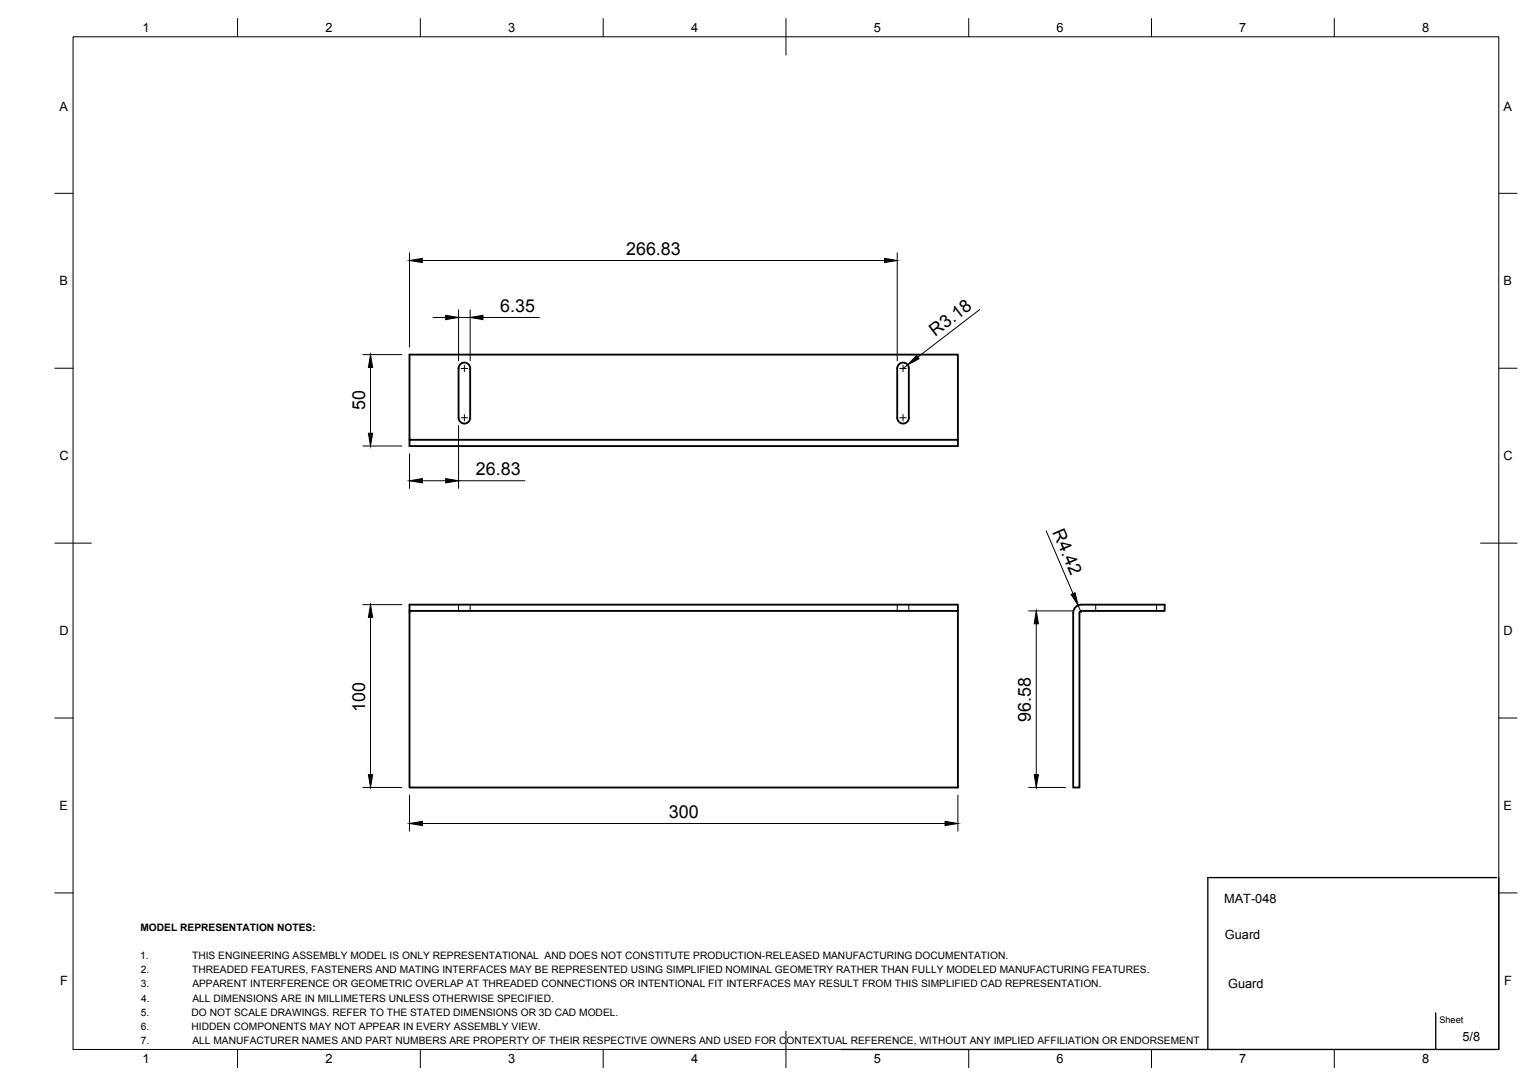
ISO-10303-21;
HEADER;
/* Generated by software containing ST-Developer
 * from STEP Tools, Inc. (www.steptools.com) 
 */

FILE_DESCRIPTION(
/* description */ ('STEP AP214'),
/* implementation_level */ '2;1');

FILE_NAME(
/* name */ 'Guard.step',
/* time_stamp */ '2026-11-14T22:24:45-08:00',
/* author */ (''),
/* organization */ (''),
/* preprocessor_version */ 'ST-DEVELOPER v20.2',
/* originating_system */ 'Autodesk Translation Framework v15.17.0.0',
/* authorisation */ '');

FILE_SCHEMA (('AUTOMOTIVE_DESIGN { 1 0 10303 214 3 1 1 }'));
ENDSEC;

DATA;
#10=MECHANICAL_DESIGN_GEOMETRIC_PRESENTATION_REPRESENTATION('',(#128),#5599);
#103=FACE_BOUND('',#588,.T.);
#104=FACE_BOUND('',#589,.T.);
#105=FACE_BOUND('',#592,.T.);
#106=FACE_BOUND('',#593,.T.);
#116=SHAPE_REPRESENTATION_RELATIONSHIP('SRR','None',#5644,#122);
#122=ADVANCED_BREP_SHAPE_REPRESENTATION('',(#134),#5596);
#128=STYLED_ITEM('',(#5680),#134);
#134=MANIFOLD_SOLID_BREP('Body1',#3310);
#171=CYLINDRICAL_SURFACE('',#3578,4.42);
#172=CYLINDRICAL_SURFACE('',#3582,1.);
#173=CYLINDRICAL_SURFACE('',#3585,3.17500000000003);
#174=CYLINDRICAL_SURFACE('',#3587,3.17500000000002);
#175=CYLINDRICAL_SURFACE('',#3589,3.17500000000004);
#176=CYLINDRICAL_SURFACE('',#3591,3.17500000000004);
#237=CIRCLE('',#3560,4.42);
#238=CIRCLE('',#3561,1.);
#239=CIRCLE('',#3564,4.42);
#240=CIRCLE('',#3565,1.);
#241=CIRCLE('',#3568,3.17500000000004);
#242=CIRCLE('',#3569,3.17500000000004);
#243=CIRCLE('',#3570,3.17500000000003);
#244=CIRCLE('',#3571,3.17500000000002);
#245=CIRCLE('',#3574,3.17500000000004);
#246=CIRCLE('',#3575,3.17500000000004);
#247=CIRCLE('',#3576,3.17500000000003);
#248=CIRCLE('',#3577,3.17500000000002);
#403=FACE_OUTER_BOUND('',#583,.T.);
#404=FACE_OUTER_BOUND('',#584,.T.);
#405=FACE_OUTER_BOUND('',#585,.T.);
#406=FACE_OUTER_BOUND('',#586,.T.);
#407=FACE_OUTER_BOUND('',#587,.T.);
#408=FACE_OUTER_BOUND('',#590,.T.);
#409=FACE_OUTER_BOUND('',#591,.T.);
#410=FACE_OUTER_BOUND('',#594,.T.);
#411=FACE_OUTER_BOUND('',#595,.T.);
#412=FACE_OUTER_BOUND('',#596,.T.);
#413=FACE_OUTER_BOUND('',#597,.T.);
#414=FACE_OUTER_BOUND('',#598,.T.);
#415=FACE_OUTER_BOUND('',#599,.T.);
#416=FACE_OUTER_BOUND('',#600,.T.);
#417=FACE_OUTER_BOUND('',#601,.T.);
#418=FACE_OUTER_BOUND('',#602,.T.);
#419=FACE_OUTER_BOUND('',#603,.T.);
#420=FACE_OUTER_BOUND('',#604,.T.);
#421=FACE_OUTER_BOUND('',#605,.T.);
#422=FACE_OUTER_BOUND('',#606,.T.);
#423=FACE_OUTER_BOUND('',#607,.T.);
#424=FACE_OUTER_BOUND('',#608,.T.);
#583=EDGE_LOOP('',(#2731,#2732,#2733,#2734));
#584=EDGE_LOOP('',(#2735,#2736,#2737,#2738));
#585=EDGE_LOOP('',(#2739,#2740,#2741,#2742));
#586=EDGE_LOOP('',(#2743,#2744,#2745,#2746));
#587=EDGE_LOOP('',(#2747,#2748,#2749,#2750));
#588=EDGE_LOOP('',(#2751,#2752,#2753,#2754));
#589=EDGE_LOOP('',(#2755,#2756,#2757,#2758));
#590=EDGE_LOOP('',(#2759,#2760,#2761,#2762));
#591=EDGE_LOOP('',(#2763,#2764,#2765,#2766));
#592=EDGE_LOOP('',(#2767,#2768,#2769,#2770));
#593=EDGE_LOOP('',(#2771,#2772,#2773,#2774));
#594=EDGE_LOOP('',(#2775,#2776,#2777,#2778));
#595=EDGE_LOOP('',(#2779,#2780,#2781,#2782));
#596=EDGE_LOOP('',(#2783,#2784,#2785,#2786));
#597=EDGE_LOOP('',(#2787,#2788,#2789,#2790));
#598=EDGE_LOOP('',(#2791,#2792,#2793,#2794));
#599=EDGE_LOOP('',(#2795,#2796,#2797,#2798));
#600=EDGE_LOOP('',(#2799,#2800,#2801,#2802));
#601=EDGE_LOOP('',(#2803,#2804,#2805,#2806));
#602=EDGE_LOOP('',(#2807,#2808,#2809,#2810));
#603=EDGE_LOOP('',(#2811,#2812,#2813,#2814));
#604=EDGE_LOOP('',(#2815,#2816,#2817,#2818));
#605=EDGE_LOOP('',(#2819,#2820,#2821,#2822));
#606=EDGE_LOOP('',(#2823,#2824,#2825,#2826));
#607=EDGE_LOOP('',(#2827,#2828,#2829,#2830));
#608=EDGE_LOOP('',(#2831,#2832,#2833,#2834));
#911=LINE('',#5285,#1267);
#912=LINE('',#5289,#1268);
#913=LINE('',#5293,#1269);
#914=LINE('',#5295,#1270);
#915=LINE('',#5296,#1271);
#916=LINE('',#5300,#1272);
#917=LINE('',#5304,#1273);
#918=LINE('',#5308,#1274);
#919=LINE('',#5310,#1275);
#920=LINE('',#5311,#1276);
#921=LINE('',#5314,#1277);
#922=LINE('',#5315,#1278);
#923=LINE('',#5316,#1279);
#924=LINE('',#5319,#1280);
#925=LINE('',#5323,#1281);
#926=LINE('',#5327,#1282);
#927=LINE('',#5331,#1283);
#928=LINE('',#5335,#1284);
#929=LINE('',#5336,#1285);
#930=LINE('',#5338,#1286);
#931=LINE('',#5339,#1287);
#932=LINE('',#5344,#1288);
#933=LINE('',#5347,#1289);
#934=LINE('',#5352,#1290);
#935=LINE('',#5355,#1291);
#936=LINE('',#5357,#1292);
#937=LINE('',#5360,#1293);
#938=LINE('',#5361,#1294);
#939=LINE('',#5364,#1295);
#940=LINE('',#5365,#1296);
#941=LINE('',#5367,#1297);
#942=LINE('',#5368,#1298);
#943=LINE('',#5373,#1299);
#944=LINE('',#5374,#1300);
#945=LINE('',#5376,#1301);
#946=LINE('',#5378,#1302);
#947=LINE('',#5381,#1303);
#948=LINE('',#5382,#1304);
#949=LINE('',#5384,#1305);
#950=LINE('',#5386,#1306);
#1267=VECTOR('',#4305,1000.);
#1268=VECTOR('',#4308,1000.);
#1269=VECTOR('',#4313,1000.);
#1270=VECTOR('',#4314,1000.);
#1271=VECTOR('',#4315,1000.);
#1272=VECTOR('',#4318,1000.);
#1273=VECTOR('',#4321,1000.);
#1274=VECTOR('',#4326,1000.);
#1275=VECTOR('',#4327,1000.);
#1276=VECTOR('',#4328,1000.);
#1277=VECTOR('',#4331,1000.);
#1278=VECTOR('',#4332,1000.);
#1279=VECTOR('',#4333,1000.);
#1280=VECTOR('',#4334,1000.);
#1281=VECTOR('',#4337,1000.);
#1282=VECTOR('',#4340,1000.);
#1283=VECTOR('',#4343,1000.);
#1284=VECTOR('',#4348,1000.);
#1285=VECTOR('',#4349,1000.);
#1286=VECTOR('',#4352,1000.);
#1287=VECTOR('',#4353,1000.);
#1288=VECTOR('',#4356,1000.);
#1289=VECTOR('',#4359,1000.);
#1290=VECTOR('',#4362,1000.);
#1291=VECTOR('',#4365,1000.);
#1292=VECTOR('',#4368,1000.);
#1293=VECTOR('',#4371,1000.);
#1294=VECTOR('',#4372,1000.);
#1295=VECTOR('',#4375,1000.);
#1296=VECTOR('',#4376,1000.);
#1297=VECTOR('',#4379,1000.);
#1298=VECTOR('',#4380,1000.);
#1299=VECTOR('',#4389,1000.);
#1300=VECTOR('',#4390,1000.);
#1301=VECTOR('',#4393,1000.);
#1302=VECTOR('',#4396,1000.);
#1303=VECTOR('',#4401,1000.);
#1304=VECTOR('',#4402,1000.);
#1305=VECTOR('',#4405,1000.);
#1306=VECTOR('',#4408,1000.);
#1559=VERTEX_POINT('',#5283);
#1560=VERTEX_POINT('',#5284);
#1561=VERTEX_POINT('',#5286);
#1562=VERTEX_POINT('',#5288);
#1563=VERTEX_POINT('',#5292);
#1564=VERTEX_POINT('',#5294);
#1565=VERTEX_POINT('',#5298);
#1566=VERTEX_POINT('',#5299);
#1567=VERTEX_POINT('',#5301);
#1568=VERTEX_POINT('',#5303);
#1569=VERTEX_POINT('',#5307);
#1570=VERTEX_POINT('',#5309);
#1571=VERTEX_POINT('',#5313);
#1572=VERTEX_POINT('',#5317);
#1573=VERTEX_POINT('',#5318);
#1574=VERTEX_POINT('',#5320);
#1575=VERTEX_POINT('',#5322);
#1576=VERTEX_POINT('',#5325);
#1577=VERTEX_POINT('',#5326);
#1578=VERTEX_POINT('',#5328);
#1579=VERTEX_POINT('',#5330);
#1580=VERTEX_POINT('',#5334);
#1581=VERTEX_POINT('',#5340);
#1582=VERTEX_POINT('',#5341);
#1583=VERTEX_POINT('',#5343);
#1584=VERTEX_POINT('',#5345);
#1585=VERTEX_POINT('',#5348);
#1586=VERTEX_POINT('',#5349);
#1587=VERTEX_POINT('',#5351);
#1588=VERTEX_POINT('',#5353);
#1589=VERTEX_POINT('',#5359);
#1590=VERTEX_POINT('',#5363);
#1963=EDGE_CURVE('',#1559,#1560,#911,.T.);
#1964=EDGE_CURVE('',#1561,#1559,#237,.T.);
#1965=EDGE_CURVE('',#1562,#1561,#912,.T.);
#1966=EDGE_CURVE('',#1562,#1560,#238,.T.);
#1967=EDGE_CURVE('',#1559,#1563,#913,.T.);
#1968=EDGE_CURVE('',#1560,#1564,#914,.T.);
#1969=EDGE_CURVE('',#1563,#1564,#915,.T.);
#1970=EDGE_CURVE('',#1565,#1566,#916,.T.);
#1971=EDGE_CURVE('',#1565,#1567,#239,.T.);
#1972=EDGE_CURVE('',#1568,#1567,#917,.T.);
#1973=EDGE_CURVE('',#1566,#1568,#240,.T.);
#1974=EDGE_CURVE('',#1569,#1565,#918,.T.);
#1975=EDGE_CURVE('',#1570,#1566,#919,.T.);
#1976=EDGE_CURVE('',#1570,#1569,#920,.T.);
#1977=EDGE_CURVE('',#1568,#1571,#921,.T.);
#1978=EDGE_CURVE('',#1564,#1571,#922,.T.);
#1979=EDGE_CURVE('',#1560,#1568,#923,.T.);
#1980=EDGE_CURVE('',#1572,#1573,#924,.T.);
#1981=EDGE_CURVE('',#1573,#1574,#241,.T.);
#1982=EDGE_CURVE('',#1574,#1575,#925,.T.);
#1983=EDGE_CURVE('',#1575,#1572,#242,.T.);
#1984=EDGE_CURVE('',#1576,#1577,#926,.T.);
#1985=EDGE_CURVE('',#1577,#1578,#243,.T.);
#1986=EDGE_CURVE('',#1578,#1579,#927,.T.);
#1987=EDGE_CURVE('',#1579,#1576,#244,.T.);
#1988=EDGE_CURVE('',#1580,#1571,#928,.T.);
#1989=EDGE_CURVE('',#1563,#1580,#929,.T.);
#1990=EDGE_CURVE('',#1567,#1580,#930,.T.);
#1991=EDGE_CURVE('',#1559,#1567,#931,.T.);
#1992=EDGE_CURVE('',#1581,#1582,#245,.T.);
#1993=EDGE_CURVE('',#1583,#1581,#932,.T.);
#1994=EDGE_CURVE('',#1584,#1583,#246,.T.);
#1995=EDGE_CURVE('',#1582,#1584,#933,.T.);
#1996=EDGE_CURVE('',#1585,#1586,#247,.T.);
#1997=EDGE_CURVE('',#1587,#1585,#934,.T.);
#1998=EDGE_CURVE('',#1588,#1587,#248,.T.);
#1999=EDGE_CURVE('',#1586,#1588,#935,.T.);
#2000=EDGE_CURVE('',#1561,#1565,#936,.T.);
#2001=EDGE_CURVE('',#1589,#1569,#937,.T.);
#2002=EDGE_CURVE('',#1589,#1561,#938,.T.);
#2003=EDGE_CURVE('',#1590,#1570,#939,.T.);
#2004=EDGE_CURVE('',#1590,#1589,#940,.T.);
#2005=EDGE_CURVE('',#1562,#1566,#941,.T.);
#2006=EDGE_CURVE('',#1590,#1562,#942,.T.);
#2007=EDGE_CURVE('',#1577,#1585,#943,.T.);
#2008=EDGE_CURVE('',#1578,#1586,#944,.T.);
#2009=EDGE_CURVE('',#1576,#1587,#945,.T.);
#2010=EDGE_CURVE('',#1579,#1588,#946,.T.);
#2011=EDGE_CURVE('',#1573,#1581,#947,.T.);
#2012=EDGE_CURVE('',#1574,#1582,#948,.T.);
#2013=EDGE_CURVE('',#1572,#1583,#949,.T.);
#2014=EDGE_CURVE('',#1575,#1584,#950,.T.);
#2731=ORIENTED_EDGE('',*,*,#1963,.F.);
#2732=ORIENTED_EDGE('',*,*,#1964,.F.);
#2733=ORIENTED_EDGE('',*,*,#1965,.F.);
#2734=ORIENTED_EDGE('',*,*,#1966,.T.);
#2735=ORIENTED_EDGE('',*,*,#1967,.F.);
#2736=ORIENTED_EDGE('',*,*,#1963,.T.);
#2737=ORIENTED_EDGE('',*,*,#1968,.T.);
#2738=ORIENTED_EDGE('',*,*,#1969,.F.);
#2739=ORIENTED_EDGE('',*,*,#1970,.F.);
#2740=ORIENTED_EDGE('',*,*,#1971,.T.);
#2741=ORIENTED_EDGE('',*,*,#1972,.F.);
#2742=ORIENTED_EDGE('',*,*,#1973,.F.);
#2743=ORIENTED_EDGE('',*,*,#1974,.T.);
#2744=ORIENTED_EDGE('',*,*,#1970,.T.);
#2745=ORIENTED_EDGE('',*,*,#1975,.F.);
#2746=ORIENTED_EDGE('',*,*,#1976,.T.);
#2747=ORIENTED_EDGE('',*,*,#1977,.T.);
#2748=ORIENTED_EDGE('',*,*,#1978,.F.);
#2749=ORIENTED_EDGE('',*,*,#1968,.F.);
#2750=ORIENTED_EDGE('',*,*,#1979,.T.);
#2751=ORIENTED_EDGE('',*,*,#1980,.T.);
#2752=ORIENTED_EDGE('',*,*,#1981,.T.);
#2753=ORIENTED_EDGE('',*,*,#1982,.T.);
#2754=ORIENTED_EDGE('',*,*,#1983,.T.);
#2755=ORIENTED_EDGE('',*,*,#1984,.T.);
#2756=ORIENTED_EDGE('',*,*,#1985,.T.);
#2757=ORIENTED_EDGE('',*,*,#1986,.T.);
#2758=ORIENTED_EDGE('',*,*,#1987,.T.);
#2759=ORIENTED_EDGE('',*,*,#1988,.F.);
#2760=ORIENTED_EDGE('',*,*,#1989,.F.);
#2761=ORIENTED_EDGE('',*,*,#1969,.T.);
#2762=ORIENTED_EDGE('',*,*,#1978,.T.);
#2763=ORIENTED_EDGE('',*,*,#1990,.F.);
#2764=ORIENTED_EDGE('',*,*,#1991,.F.);
#2765=ORIENTED_EDGE('',*,*,#1967,.T.);
#2766=ORIENTED_EDGE('',*,*,#1989,.T.);
#2767=ORIENTED_EDGE('',*,*,#1992,.F.);
#2768=ORIENTED_EDGE('',*,*,#1993,.F.);
#2769=ORIENTED_EDGE('',*,*,#1994,.F.);
#2770=ORIENTED_EDGE('',*,*,#1995,.F.);
#2771=ORIENTED_EDGE('',*,*,#1996,.F.);
#2772=ORIENTED_EDGE('',*,*,#1997,.F.);
#2773=ORIENTED_EDGE('',*,*,#1998,.F.);
#2774=ORIENTED_EDGE('',*,*,#1999,.F.);
#2775=ORIENTED_EDGE('',*,*,#1971,.F.);
#2776=ORIENTED_EDGE('',*,*,#2000,.F.);
#2777=ORIENTED_EDGE('',*,*,#1964,.T.);
#2778=ORIENTED_EDGE('',*,*,#1991,.T.);
#2779=ORIENTED_EDGE('',*,*,#1974,.F.);
#2780=ORIENTED_EDGE('',*,*,#2001,.F.);
#2781=ORIENTED_EDGE('',*,*,#2002,.T.);
#2782=ORIENTED_EDGE('',*,*,#2000,.T.);
#2783=ORIENTED_EDGE('',*,*,#1976,.F.);
#2784=ORIENTED_EDGE('',*,*,#2003,.F.);
#2785=ORIENTED_EDGE('',*,*,#2004,.T.);
#2786=ORIENTED_EDGE('',*,*,#2001,.T.);
#2787=ORIENTED_EDGE('',*,*,#1975,.T.);
#2788=ORIENTED_EDGE('',*,*,#2005,.F.);
#2789=ORIENTED_EDGE('',*,*,#2006,.F.);
#2790=ORIENTED_EDGE('',*,*,#2003,.T.);
#2791=ORIENTED_EDGE('',*,*,#1973,.T.);
#2792=ORIENTED_EDGE('',*,*,#1979,.F.);
#2793=ORIENTED_EDGE('',*,*,#1966,.F.);
#2794=ORIENTED_EDGE('',*,*,#2005,.T.);
#2795=ORIENTED_EDGE('',*,*,#2006,.T.);
#2796=ORIENTED_EDGE('',*,*,#1965,.T.);
#2797=ORIENTED_EDGE('',*,*,#2002,.F.);
#2798=ORIENTED_EDGE('',*,*,#2004,.F.);
#2799=ORIENTED_EDGE('',*,*,#1977,.F.);
#2800=ORIENTED_EDGE('',*,*,#1972,.T.);
#2801=ORIENTED_EDGE('',*,*,#1990,.T.);
#2802=ORIENTED_EDGE('',*,*,#1988,.T.);
#2803=ORIENTED_EDGE('',*,*,#2007,.T.);
#2804=ORIENTED_EDGE('',*,*,#1996,.T.);
#2805=ORIENTED_EDGE('',*,*,#2008,.F.);
#2806=ORIENTED_EDGE('',*,*,#1985,.F.);
#2807=ORIENTED_EDGE('',*,*,#2009,.T.);
#2808=ORIENTED_EDGE('',*,*,#1997,.T.);
#2809=ORIENTED_EDGE('',*,*,#2007,.F.);
#2810=ORIENTED_EDGE('',*,*,#1984,.F.);
#2811=ORIENTED_EDGE('',*,*,#2010,.T.);
#2812=ORIENTED_EDGE('',*,*,#1998,.T.);
#2813=ORIENTED_EDGE('',*,*,#2009,.F.);
#2814=ORIENTED_EDGE('',*,*,#1987,.F.);
#2815=ORIENTED_EDGE('',*,*,#2008,.T.);
#2816=ORIENTED_EDGE('',*,*,#1999,.T.);
#2817=ORIENTED_EDGE('',*,*,#2010,.F.);
#2818=ORIENTED_EDGE('',*,*,#1986,.F.);
#2819=ORIENTED_EDGE('',*,*,#2011,.T.);
#2820=ORIENTED_EDGE('',*,*,#1992,.T.);
#2821=ORIENTED_EDGE('',*,*,#2012,.F.);
#2822=ORIENTED_EDGE('',*,*,#1981,.F.);
#2823=ORIENTED_EDGE('',*,*,#2013,.T.);
#2824=ORIENTED_EDGE('',*,*,#1993,.T.);
#2825=ORIENTED_EDGE('',*,*,#2011,.F.);
#2826=ORIENTED_EDGE('',*,*,#1980,.F.);
#2827=ORIENTED_EDGE('',*,*,#2014,.T.);
#2828=ORIENTED_EDGE('',*,*,#1994,.T.);
#2829=ORIENTED_EDGE('',*,*,#2013,.F.);
#2830=ORIENTED_EDGE('',*,*,#1983,.F.);
#2831=ORIENTED_EDGE('',*,*,#2012,.T.);
#2832=ORIENTED_EDGE('',*,*,#1995,.T.);
#2833=ORIENTED_EDGE('',*,*,#2014,.F.);
#2834=ORIENTED_EDGE('',*,*,#1982,.F.);
#3099=PLANE('',#3559);
#3100=PLANE('',#3562);
#3101=PLANE('',#3563);
#3102=PLANE('',#3566);
#3103=PLANE('',#3567);
#3104=PLANE('',#3572);
#3105=PLANE('',#3573);
#3106=PLANE('',#3579);
#3107=PLANE('',#3580);
#3108=PLANE('',#3581);
#3109=PLANE('',#3583);
#3110=PLANE('',#3584);
#3111=PLANE('',#3586);
#3112=PLANE('',#3588);
#3113=PLANE('',#3590);
#3114=PLANE('',#3592);
#3253=ADVANCED_FACE('',(#403),#3099,.T.);
#3254=ADVANCED_FACE('',(#404),#3100,.T.);
#3255=ADVANCED_FACE('',(#405),#3101,.T.);
#3256=ADVANCED_FACE('',(#406),#3102,.T.);
#3257=ADVANCED_FACE('',(#407,#103,#104),#3103,.F.);
#3258=ADVANCED_FACE('',(#408),#3104,.T.);
#3259=ADVANCED_FACE('',(#409,#105,#106),#3105,.T.);
#3260=ADVANCED_FACE('',(#410),#171,.T.);
#3261=ADVANCED_FACE('',(#411),#3106,.T.);
#3262=ADVANCED_FACE('',(#412),#3107,.T.);
#3263=ADVANCED_FACE('',(#413),#3108,.F.);
#3264=ADVANCED_FACE('',(#414),#172,.F.);
#3265=ADVANCED_FACE('',(#415),#3109,.T.);
#3266=ADVANCED_FACE('',(#416),#3110,.F.);
#3267=ADVANCED_FACE('',(#417),#173,.F.);
#3268=ADVANCED_FACE('',(#418),#3111,.F.);
#3269=ADVANCED_FACE('',(#419),#174,.F.);
#3270=ADVANCED_FACE('',(#420),#3112,.F.);
#3271=ADVANCED_FACE('',(#421),#175,.F.);
#3272=ADVANCED_FACE('',(#422),#3113,.F.);
#3273=ADVANCED_FACE('',(#423),#176,.F.);
#3274=ADVANCED_FACE('',(#424),#3114,.F.);
#3310=CLOSED_SHELL('',(#3253,#3254,#3255,#3256,#3257,#3258,#3259,#3260,
#3261,#3262,#3263,#3264,#3265,#3266,#3267,#3268,#3269,#3270,#3271,#3272,
#3273,#3274));
#3558=AXIS2_PLACEMENT_3D('',#5281,#4301,#4302);
#3559=AXIS2_PLACEMENT_3D('',#5282,#4303,#4304);
#3560=AXIS2_PLACEMENT_3D('',#5287,#4306,#4307);
#3561=AXIS2_PLACEMENT_3D('',#5290,#4309,#4310);
#3562=AXIS2_PLACEMENT_3D('',#5291,#4311,#4312);
#3563=AXIS2_PLACEMENT_3D('',#5297,#4316,#4317);
#3564=AXIS2_PLACEMENT_3D('',#5302,#4319,#4320);
#3565=AXIS2_PLACEMENT_3D('',#5305,#4322,#4323);
#3566=AXIS2_PLACEMENT_3D('',#5306,#4324,#4325);
#3567=AXIS2_PLACEMENT_3D('',#5312,#4329,#4330);
#3568=AXIS2_PLACEMENT_3D('',#5321,#4335,#4336);
#3569=AXIS2_PLACEMENT_3D('',#5324,#4338,#4339);
#3570=AXIS2_PLACEMENT_3D('',#5329,#4341,#4342);
#3571=AXIS2_PLACEMENT_3D('',#5332,#4344,#4345);
#3572=AXIS2_PLACEMENT_3D('',#5333,#4346,#4347);
#3573=AXIS2_PLACEMENT_3D('',#5337,#4350,#4351);
#3574=AXIS2_PLACEMENT_3D('',#5342,#4354,#4355);
#3575=AXIS2_PLACEMENT_3D('',#5346,#4357,#4358);
#3576=AXIS2_PLACEMENT_3D('',#5350,#4360,#4361);
#3577=AXIS2_PLACEMENT_3D('',#5354,#4363,#4364);
#3578=AXIS2_PLACEMENT_3D('',#5356,#4366,#4367);
#3579=AXIS2_PLACEMENT_3D('',#5358,#4369,#4370);
#3580=AXIS2_PLACEMENT_3D('',#5362,#4373,#4374);
#3581=AXIS2_PLACEMENT_3D('',#5366,#4377,#4378);
#3582=AXIS2_PLACEMENT_3D('',#5369,#4381,#4382);
#3583=AXIS2_PLACEMENT_3D('',#5370,#4383,#4384);
#3584=AXIS2_PLACEMENT_3D('',#5371,#4385,#4386);
#3585=AXIS2_PLACEMENT_3D('',#5372,#4387,#4388);
#3586=AXIS2_PLACEMENT_3D('',#5375,#4391,#4392);
#3587=AXIS2_PLACEMENT_3D('',#5377,#4394,#4395);
#3588=AXIS2_PLACEMENT_3D('',#5379,#4397,#4398);
#3589=AXIS2_PLACEMENT_3D('',#5380,#4399,#4400);
#3590=AXIS2_PLACEMENT_3D('',#5383,#4403,#4404);
#3591=AXIS2_PLACEMENT_3D('',#5385,#4406,#4407);
#3592=AXIS2_PLACEMENT_3D('',#5387,#4409,#4410);
#4301=DIRECTION('axis',(0.,0.,1.));
#4302=DIRECTION('refdir',(1.,0.,0.));
#4303=DIRECTION('center_axis',(0.,0.,1.));
#4304=DIRECTION('ref_axis',(1.,0.,0.));
#4305=DIRECTION('',(0.,-1.,0.));
#4306=DIRECTION('center_axis',(0.,0.,-1.));
#4307=DIRECTION('ref_axis',(1.,0.,0.));
#4308=DIRECTION('',(-1.,-1.21734980770302E-14,0.));
#4309=DIRECTION('center_axis',(0.,0.,-1.));
#4310=DIRECTION('ref_axis',(1.,0.,0.));
#4311=DIRECTION('center_axis',(0.,0.,1.));
#4312=DIRECTION('ref_axis',(1.,0.,0.));
#4313=DIRECTION('',(1.,0.,0.));
#4314=DIRECTION('',(1.,0.,0.));
#4315=DIRECTION('',(0.,-1.,0.));
#4316=DIRECTION('center_axis',(0.,0.,-1.));
#4317=DIRECTION('ref_axis',(-1.,0.,0.));
#4318=DIRECTION('',(1.,1.21734980770302E-14,0.));
#4319=DIRECTION('center_axis',(0.,0.,-1.));
#4320=DIRECTION('ref_axis',(1.,0.,0.));
#4321=DIRECTION('',(0.,1.,0.));
#4322=DIRECTION('center_axis',(0.,0.,-1.));
#4323=DIRECTION('ref_axis',(1.,0.,0.));
#4324=DIRECTION('center_axis',(0.,0.,-1.));
#4325=DIRECTION('ref_axis',(-1.,0.,0.));
#4326=DIRECTION('',(0.,1.,0.));
#4327=DIRECTION('',(0.,1.,0.));
#4328=DIRECTION('',(-1.,0.,0.));
#4329=DIRECTION('center_axis',(0.,1.,0.));
#4330=DIRECTION('ref_axis',(0.,0.,1.));
#4331=DIRECTION('',(1.,0.,0.));
#4332=DIRECTION('',(0.,0.,-1.));
#4333=DIRECTION('',(0.,0.,-1.));
#4334=DIRECTION('',(1.,0.,0.));
#4335=DIRECTION('center_axis',(0.,1.,0.));
#4336=DIRECTION('ref_axis',(0.,0.,1.));
#4337=DIRECTION('',(-1.,0.,0.));
#4338=DIRECTION('center_axis',(0.,1.,0.));
#4339=DIRECTION('ref_axis',(0.,0.,1.));
#4340=DIRECTION('',(1.,0.,0.));
#4341=DIRECTION('center_axis',(0.,1.,0.));
#4342=DIRECTION('ref_axis',(0.,0.,1.));
#4343=DIRECTION('',(-1.,0.,5.14311353474695E-16));
#4344=DIRECTION('center_axis',(0.,1.,0.));
#4345=DIRECTION('ref_axis',(0.,0.,1.));
#4346=DIRECTION('center_axis',(1.,0.,0.));
#4347=DIRECTION('ref_axis',(0.,0.,-1.));
#4348=DIRECTION('',(0.,-1.,0.));
#4349=DIRECTION('',(0.,0.,-1.));
#4350=DIRECTION('center_axis',(0.,1.,0.));
#4351=DIRECTION('ref_axis',(0.,0.,1.));
#4352=DIRECTION('',(1.,0.,0.));
#4353=DIRECTION('',(0.,0.,-1.));
#4354=DIRECTION('center_axis',(0.,1.,0.));
#4355=DIRECTION('ref_axis',(0.,0.,1.));
#4356=DIRECTION('',(1.,0.,0.));
#4357=DIRECTION('center_axis',(0.,1.,0.));
#4358=DIRECTION('ref_axis',(0.,0.,1.));
#4359=DIRECTION('',(-1.,0.,0.));
#4360=DIRECTION('center_axis',(0.,1.,0.));
#4361=DIRECTION('ref_axis',(0.,0.,-1.));
#4362=DIRECTION('',(1.,0.,0.));
#4363=DIRECTION('center_axis',(0.,1.,0.));
#4364=DIRECTION('ref_axis',(0.,0.,-1.));
#4365=DIRECTION('',(-1.,0.,5.14311353474694E-16));
#4366=DIRECTION('center_axis',(0.,0.,-1.));
#4367=DIRECTION('ref_axis',(-1.,0.,0.));
#4368=DIRECTION('',(0.,0.,-1.));
#4369=DIRECTION('center_axis',(-1.,0.,0.));
#4370=DIRECTION('ref_axis',(0.,0.,1.));
#4371=DIRECTION('',(0.,0.,-1.));
#4372=DIRECTION('',(0.,1.,0.));
#4373=DIRECTION('center_axis',(0.,-1.,0.));
#4374=DIRECTION('ref_axis',(0.,0.,-1.));
#4375=DIRECTION('',(0.,0.,-1.));
#4376=DIRECTION('',(-1.,0.,0.));
#4377=DIRECTION('center_axis',(-1.,0.,0.));
#4378=DIRECTION('ref_axis',(0.,0.,1.));
#4379=DIRECTION('',(0.,0.,-1.));
#4380=DIRECTION('',(0.,1.,0.));
#4381=DIRECTION('center_axis',(0.,0.,-1.));
#4382=DIRECTION('ref_axis',(-1.,0.,0.));
#4383=DIRECTION('center_axis',(0.,0.,1.));
#4384=DIRECTION('ref_axis',(1.,0.,0.));
#4385=DIRECTION('center_axis',(0.,0.,1.));
#4386=DIRECTION('ref_axis',(1.,0.,0.));
#4387=DIRECTION('center_axis',(0.,1.,0.));
#4388=DIRECTION('ref_axis',(0.,0.,1.));
#4389=DIRECTION('',(0.,1.,0.));
#4390=DIRECTION('',(0.,1.,0.));
#4391=DIRECTION('center_axis',(0.,0.,1.));
#4392=DIRECTION('ref_axis',(1.,0.,0.));
#4393=DIRECTION('',(0.,1.,0.));
#4394=DIRECTION('center_axis',(0.,1.,0.));
#4395=DIRECTION('ref_axis',(0.,0.,1.));
#4396=DIRECTION('',(0.,1.,0.));
#4397=DIRECTION('center_axis',(-5.14311353474695E-16,0.,-1.));
#4398=DIRECTION('ref_axis',(-1.,0.,5.14311353474695E-16));
#4399=DIRECTION('center_axis',(0.,1.,0.));
#4400=DIRECTION('ref_axis',(0.,0.,1.));
#4401=DIRECTION('',(0.,1.,0.));
#4402=DIRECTION('',(0.,1.,0.));
#4403=DIRECTION('center_axis',(0.,0.,1.));
#4404=DIRECTION('ref_axis',(1.,0.,0.));
#4405=DIRECTION('',(0.,1.,0.));
#4406=DIRECTION('center_axis',(0.,1.,0.));
#4407=DIRECTION('ref_axis',(0.,0.,1.));
#4408=DIRECTION('',(0.,1.,0.));
#4409=DIRECTION('center_axis',(0.,0.,-1.));
#4410=DIRECTION('ref_axis',(-1.,0.,0.));
#5281=CARTESIAN_POINT('',(0.,0.,0.));
#5282=CARTESIAN_POINT('Origin',(4.42,100.,300.));
#5283=CARTESIAN_POINT('',(4.42,100.,300.));
#5284=CARTESIAN_POINT('',(4.42,96.58,300.));
#5285=CARTESIAN_POINT('',(4.42,100.,300.));
#5286=CARTESIAN_POINT('',(0.,95.5799999999999,300.));
#5287=CARTESIAN_POINT('Origin',(4.42,95.58,300.));
#5288=CARTESIAN_POINT('',(3.42,95.58,300.));
#5289=CARTESIAN_POINT('',(3.42,95.58,300.));
#5290=CARTESIAN_POINT('Origin',(4.42,95.58,300.));
#5291=CARTESIAN_POINT('Origin',(3.42,95.58,300.));
#5292=CARTESIAN_POINT('',(50.,100.,300.));
#5293=CARTESIAN_POINT('',(0.,100.,300.));
#5294=CARTESIAN_POINT('',(50.,96.58,300.));
#5295=CARTESIAN_POINT('',(0.,96.58,300.));
#5296=CARTESIAN_POINT('',(50.,100.,300.));
#5297=CARTESIAN_POINT('Origin',(0.,95.5799999999999,0.));
#5298=CARTESIAN_POINT('',(0.,95.5799999999999,0.));
#5299=CARTESIAN_POINT('',(3.42,95.58,-5.55111512312578E-14));
#5300=CARTESIAN_POINT('',(0.,95.5799999999999,0.));
#5301=CARTESIAN_POINT('',(4.42,100.,0.));
#5302=CARTESIAN_POINT('Origin',(4.42,95.58,0.));
#5303=CARTESIAN_POINT('',(4.42,96.58,0.));
#5304=CARTESIAN_POINT('',(4.42,96.58,0.));
#5305=CARTESIAN_POINT('Origin',(4.42,95.58,0.));
#5306=CARTESIAN_POINT('Origin',(4.42,96.58,0.));
#5307=CARTESIAN_POINT('',(0.,0.,0.));
#5308=CARTESIAN_POINT('',(0.,0.,0.));
#5309=CARTESIAN_POINT('',(3.42,0.,-5.55111512312578E-14));
#5310=CARTESIAN_POINT('',(3.42,0.,-5.55111512312578E-14));
#5311=CARTESIAN_POINT('',(3.42,0.,-5.55111512312578E-14));
#5312=CARTESIAN_POINT('Origin',(0.,96.58,300.));
#5313=CARTESIAN_POINT('',(50.,96.58,-5.55111512312578E-14));
#5314=CARTESIAN_POINT('',(0.,96.58,0.));
#5315=CARTESIAN_POINT('',(50.,96.58,300.));
#5316=CARTESIAN_POINT('',(4.42,96.58,300.));
#5317=CARTESIAN_POINT('',(15.4661722120008,96.58,273.175));
#5318=CARTESIAN_POINT('',(42.4494143941068,96.58,273.175));
#5319=CARTESIAN_POINT('',(0.,96.58,273.175));
#5320=CARTESIAN_POINT('',(42.4494143941069,96.58,266.825));
#5321=CARTESIAN_POINT('Origin',(42.4494143941068,96.58,270.));
#5322=CARTESIAN_POINT('',(15.4661722120007,96.58,266.825));
#5323=CARTESIAN_POINT('',(1.38777878078145E-14,96.58,266.825));
#5324=CARTESIAN_POINT('Origin',(15.4661722120008,96.58,270.));
#5325=CARTESIAN_POINT('',(15.4661722120007,96.58,33.1749999999999));
#5326=CARTESIAN_POINT('',(42.4494143941068,96.58,33.1749999999999));
#5327=CARTESIAN_POINT('',(0.,96.58,33.1749999999999));
#5328=CARTESIAN_POINT('',(42.4494143941068,96.58,26.8249999999998));
#5329=CARTESIAN_POINT('Origin',(42.4494143941068,96.58,29.9999999999998));
#5330=CARTESIAN_POINT('',(15.4661722120007,96.58,26.8249999999998));
#5331=CARTESIAN_POINT('',(-1.38777878078145E-13,96.58,26.8249999999999));
#5332=CARTESIAN_POINT('Origin',(15.4661722120007,96.58,29.9999999999999));
#5333=CARTESIAN_POINT('Origin',(50.,100.,300.));
#5334=CARTESIAN_POINT('',(50.,100.,-5.55111512312578E-14));
#5335=CARTESIAN_POINT('',(50.,100.,-5.55111512312578E-14));
#5336=CARTESIAN_POINT('',(50.,100.,300.));
#5337=CARTESIAN_POINT('Origin',(0.,100.,300.));
#5338=CARTESIAN_POINT('',(0.,100.,0.));
#5339=CARTESIAN_POINT('',(4.42,100.,300.));
#5340=CARTESIAN_POINT('',(42.4494143941068,100.,273.175));
#5341=CARTESIAN_POINT('',(42.4494143941069,100.,266.825));
#5342=CARTESIAN_POINT('Origin',(42.4494143941068,100.,270.));
#5343=CARTESIAN_POINT('',(15.4661722120008,100.,273.175));
#5344=CARTESIAN_POINT('',(42.4494143941068,100.,273.175));
#5345=CARTESIAN_POINT('',(15.4661722120007,100.,266.825));
#5346=CARTESIAN_POINT('Origin',(15.4661722120008,100.,270.));
#5347=CARTESIAN_POINT('',(42.4494143941069,100.,266.825));
#5348=CARTESIAN_POINT('',(42.4494143941068,100.,33.1749999999999));
#5349=CARTESIAN_POINT('',(42.4494143941068,100.,26.8249999999998));
#5350=CARTESIAN_POINT('Origin',(42.4494143941068,100.,29.9999999999998));
#5351=CARTESIAN_POINT('',(15.4661722120007,100.,33.1749999999999));
#5352=CARTESIAN_POINT('',(42.4494143941068,100.,33.1749999999999));
#5353=CARTESIAN_POINT('',(15.4661722120007,100.,26.8249999999999));
#5354=CARTESIAN_POINT('Origin',(15.4661722120007,100.,29.9999999999999));
#5355=CARTESIAN_POINT('',(42.4494143941068,100.,26.8249999999998));
#5356=CARTESIAN_POINT('Origin',(4.42,95.58,300.));
#5357=CARTESIAN_POINT('',(0.,95.5799999999999,300.));
#5358=CARTESIAN_POINT('Origin',(0.,0.,300.));
#5359=CARTESIAN_POINT('',(0.,0.,300.));
#5360=CARTESIAN_POINT('',(0.,0.,300.));
#5361=CARTESIAN_POINT('',(0.,0.,300.));
#5362=CARTESIAN_POINT('Origin',(3.42,0.,300.));
#5363=CARTESIAN_POINT('',(3.42,0.,300.));
#5364=CARTESIAN_POINT('',(3.42,0.,300.));
#5365=CARTESIAN_POINT('',(3.42,0.,300.));
#5366=CARTESIAN_POINT('Origin',(3.42,0.,300.));
#5367=CARTESIAN_POINT('',(3.42,95.58,300.));
#5368=CARTESIAN_POINT('',(3.42,0.,300.));
#5369=CARTESIAN_POINT('Origin',(4.42,95.58,300.));
#5370=CARTESIAN_POINT('Origin',(4.42,95.58,300.));
#5371=CARTESIAN_POINT('Origin',(4.42,95.58,0.));
#5372=CARTESIAN_POINT('Origin',(42.4494143941068,90.,29.9999999999998));
#5373=CARTESIAN_POINT('',(42.4494143941068,90.,33.1749999999999));
#5374=CARTESIAN_POINT('',(42.4494143941068,90.,26.8249999999998));
#5375=CARTESIAN_POINT('Origin',(42.4494143941068,90.,33.1749999999999));
#5376=CARTESIAN_POINT('',(15.4661722120007,90.,33.1749999999999));
#5377=CARTESIAN_POINT('Origin',(15.4661722120007,90.,29.9999999999999));
#5378=CARTESIAN_POINT('',(15.4661722120007,90.,26.8249999999999));
#5379=CARTESIAN_POINT('Origin',(42.4494143941068,90.,26.8249999999998));
#5380=CARTESIAN_POINT('Origin',(42.4494143941068,90.,270.));
#5381=CARTESIAN_POINT('',(42.4494143941068,90.,273.175));
#5382=CARTESIAN_POINT('',(42.4494143941069,90.,266.825));
#5383=CARTESIAN_POINT('Origin',(42.4494143941068,90.,273.175));
#5384=CARTESIAN_POINT('',(15.4661722120008,90.,273.175));
#5385=CARTESIAN_POINT('Origin',(15.4661722120008,90.,270.));
#5386=CARTESIAN_POINT('',(15.4661722120007,90.,266.825));
#5387=CARTESIAN_POINT('Origin',(42.4494143941069,90.,266.825));
#5588=UNCERTAINTY_MEASURE_WITH_UNIT(LENGTH_MEASURE(0.01),#5600,
'DISTANCE_ACCURACY_VALUE',
'Maximum model space distance between geometric entities at asserted c
onnectivities');
#5591=UNCERTAINTY_MEASURE_WITH_UNIT(LENGTH_MEASURE(0.01),#5600,
'DISTANCE_ACCURACY_VALUE',
'Maximum model space distance between geometric entities at asserted c
onnectivities');
#5596=(
GEOMETRIC_REPRESENTATION_CONTEXT(3)
GLOBAL_UNCERTAINTY_ASSIGNED_CONTEXT((#5588))
GLOBAL_UNIT_ASSIGNED_CONTEXT((#5600,#5602,#5603))
REPRESENTATION_CONTEXT('','3D')
);
#5599=(
GEOMETRIC_REPRESENTATION_CONTEXT(3)
GLOBAL_UNCERTAINTY_ASSIGNED_CONTEXT((#5591))
GLOBAL_UNIT_ASSIGNED_CONTEXT((#5600,#5602,#5603))
REPRESENTATION_CONTEXT('','3D')
);
#5600=(
LENGTH_UNIT()
NAMED_UNIT(*)
SI_UNIT(.MILLI.,.METRE.)
);
#5602=(
NAMED_UNIT(*)
PLANE_ANGLE_UNIT()
SI_UNIT($,.RADIAN.)
);
#5603=(
NAMED_UNIT(*)
SI_UNIT($,.STERADIAN.)
SOLID_ANGLE_UNIT()
);
#5608=SHAPE_DEFINITION_REPRESENTATION(#5615,#5644);
#5615=PRODUCT_DEFINITION_SHAPE('',$,#5652);
#5644=SHAPE_REPRESENTATION('',(#3558),#5596);
#5647=PRODUCT_DEFINITION_CONTEXT('part definition',#5670,'design');
#5652=PRODUCT_DEFINITION('Guard','Guard',#5659,#5647);
#5659=PRODUCT_DEFINITION_FORMATION('',$,#5676);
#5670=APPLICATION_CONTEXT(
'Core Data for Automotive Mechanical Design Process');
#5671=PRODUCT_CONTEXT('part definition',#5670,'mechanical');
#5676=PRODUCT('Guard','Guard',$,(#5671));
#5680=PRESENTATION_STYLE_ASSIGNMENT((#5683));
#5683=SURFACE_STYLE_USAGE(.BOTH.,#5686);
#5686=SURFACE_SIDE_STYLE('',(#5689));
#5689=SURFACE_STYLE_FILL_AREA(#5692);
#5692=FILL_AREA_STYLE('Opaque(97,158,199)',(#5695));
#5695=FILL_AREA_STYLE_COLOUR('Opaque(97,158,199)',#5698);
#5698=COLOUR_RGB('Opaque(97,158,199)',0.380392156862745,0.619607843137255,
0.780392156862745);
ENDSEC;
END-ISO-10303-21;
